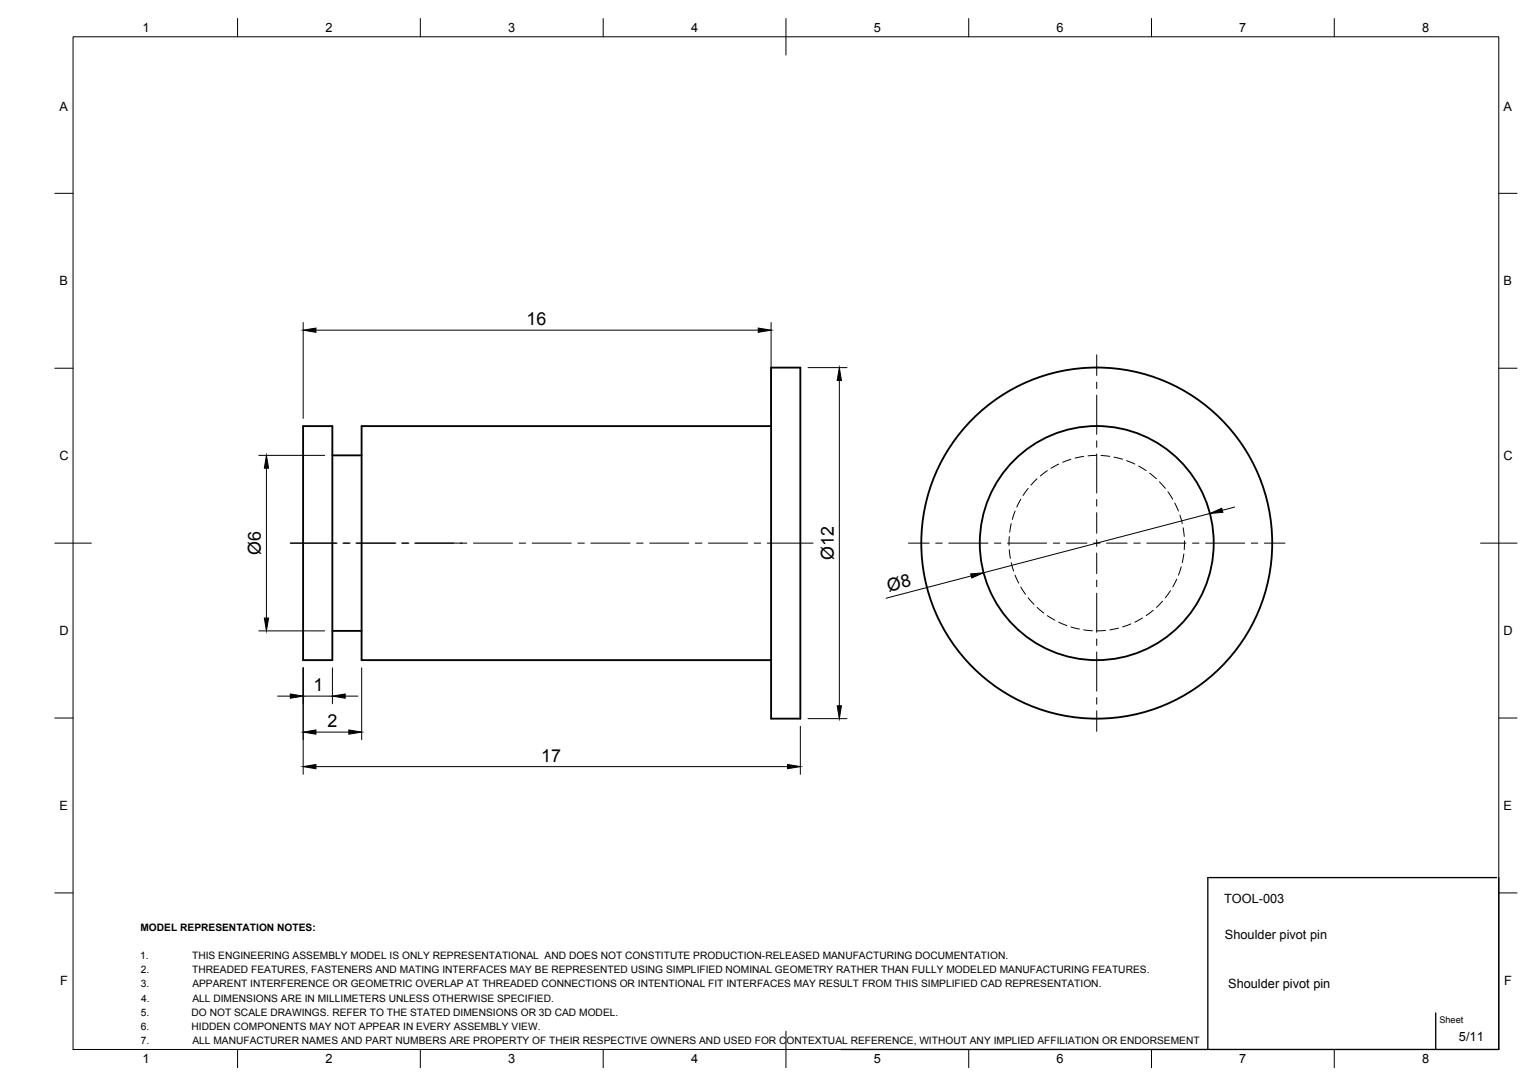
ISO-10303-21;
HEADER;
/* Generated by software containing ST-Developer
 * from STEP Tools, Inc. (www.steptools.com) 
 */

FILE_DESCRIPTION(
/* description */ (''),
/* implementation_level */ '2;1');

FILE_NAME(
/* name */ 'Shoulder pivot pin.step',
/* time_stamp */ '2026-11-10T05:20:16-08:00',
/* author */ (''),
/* organization */ (''),
/* preprocessor_version */ 'ST-DEVELOPER v20.2',
/* originating_system */ 'Autodesk Translation Framework v15.17.0.0',
/* authorisation */ '');

FILE_SCHEMA (('AUTOMOTIVE_DESIGN { 1 0 10303 214 3 1 1 }'));
ENDSEC;

DATA;
#10=MECHANICAL_DESIGN_GEOMETRIC_PRESENTATION_REPRESENTATION('',(#114),#24809);
#94=SHAPE_REPRESENTATION_RELATIONSHIP('SRR','None',#24857,#104);
#104=ADVANCED_BREP_SHAPE_REPRESENTATION('',(#124),#24800);
#114=STYLED_ITEM('',(#24920),#124);
#124=MANIFOLD_SOLID_BREP('Body1',#9891);
#144=FACE_BOUND('',#2081,.T.);
#145=FACE_BOUND('',#2083,.T.);
#146=FACE_BOUND('',#2086,.T.);
#1187=PLANE('',#10235);
#1188=PLANE('',#10237);
#1189=PLANE('',#10241);
#1190=PLANE('',#10246);
#1191=PLANE('',#10248);
#1514=FACE_OUTER_BOUND('',#2079,.T.);
#1515=FACE_OUTER_BOUND('',#2080,.T.);
#1516=FACE_OUTER_BOUND('',#2082,.T.);
#1517=FACE_OUTER_BOUND('',#2084,.T.);
#1518=FACE_OUTER_BOUND('',#2085,.T.);
#1519=FACE_OUTER_BOUND('',#2087,.T.);
#1520=FACE_OUTER_BOUND('',#2088,.T.);
#1521=FACE_OUTER_BOUND('',#2089,.T.);
#1522=FACE_OUTER_BOUND('',#2090,.T.);
#2079=EDGE_LOOP('',(#7449,#7450,#7451,#7452));
#2080=EDGE_LOOP('',(#7453));
#2081=EDGE_LOOP('',(#7454));
#2082=EDGE_LOOP('',(#7455));
#2083=EDGE_LOOP('',(#7456));
#2084=EDGE_LOOP('',(#7457,#7458,#7459,#7460));
#2085=EDGE_LOOP('',(#7461));
#2086=EDGE_LOOP('',(#7462));
#2087=EDGE_LOOP('',(#7463,#7464,#7465,#7466));
#2088=EDGE_LOOP('',(#7467));
#2089=EDGE_LOOP('',(#7468,#7469,#7470,#7471));
#2090=EDGE_LOOP('',(#7472));
#2727=LINE('',#14885,#3315);
#2728=LINE('',#14896,#3316);
#2729=LINE('',#14904,#3317);
#2730=LINE('',#14908,#3318);
#3315=VECTOR('',#11365,0.3);
#3316=VECTOR('',#11380,0.4);
#3317=VECTOR('',#11389,0.6);
#3318=VECTOR('',#11396,0.4);
#3679=CIRCLE('',#10233,0.3);
#3680=CIRCLE('',#10234,0.3);
#3681=CIRCLE('',#10236,0.4);
#3682=CIRCLE('',#10238,0.4);
#3683=CIRCLE('',#10240,0.4);
#3684=CIRCLE('',#10242,0.6);
#3685=CIRCLE('',#10243,0.4);
#3686=CIRCLE('',#10245,0.6);
#4223=VERTEX_POINT('',#14882);
#4224=VERTEX_POINT('',#14884);
#4225=VERTEX_POINT('',#14888);
#4226=VERTEX_POINT('',#14891);
#4227=VERTEX_POINT('',#14894);
#4228=VERTEX_POINT('',#14898);
#4229=VERTEX_POINT('',#14900);
#4230=VERTEX_POINT('',#14903);
#5383=EDGE_CURVE('',#4223,#4223,#3679,.T.);
#5384=EDGE_CURVE('',#4223,#4224,#2727,.T.);
#5385=EDGE_CURVE('',#4224,#4224,#3680,.T.);
#5386=EDGE_CURVE('',#4225,#4225,#3681,.T.);
#5387=EDGE_CURVE('',#4226,#4226,#3682,.T.);
#5388=EDGE_CURVE('',#4227,#4227,#3683,.T.);
#5389=EDGE_CURVE('',#4227,#4226,#2728,.T.);
#5390=EDGE_CURVE('',#4228,#4228,#3684,.T.);
#5391=EDGE_CURVE('',#4229,#4229,#3685,.T.);
#5392=EDGE_CURVE('',#4228,#4230,#2729,.T.);
#5393=EDGE_CURVE('',#4230,#4230,#3686,.T.);
#5394=EDGE_CURVE('',#4225,#4229,#2730,.T.);
#7449=ORIENTED_EDGE('',*,*,#5383,.T.);
#7450=ORIENTED_EDGE('',*,*,#5384,.T.);
#7451=ORIENTED_EDGE('',*,*,#5385,.F.);
#7452=ORIENTED_EDGE('',*,*,#5384,.F.);
#7453=ORIENTED_EDGE('',*,*,#5386,.F.);
#7454=ORIENTED_EDGE('',*,*,#5383,.F.);
#7455=ORIENTED_EDGE('',*,*,#5387,.F.);
#7456=ORIENTED_EDGE('',*,*,#5385,.T.);
#7457=ORIENTED_EDGE('',*,*,#5388,.F.);
#7458=ORIENTED_EDGE('',*,*,#5389,.T.);
#7459=ORIENTED_EDGE('',*,*,#5387,.T.);
#7460=ORIENTED_EDGE('',*,*,#5389,.F.);
#7461=ORIENTED_EDGE('',*,*,#5390,.T.);
#7462=ORIENTED_EDGE('',*,*,#5391,.F.);
#7463=ORIENTED_EDGE('',*,*,#5390,.F.);
#7464=ORIENTED_EDGE('',*,*,#5392,.T.);
#7465=ORIENTED_EDGE('',*,*,#5393,.T.);
#7466=ORIENTED_EDGE('',*,*,#5392,.F.);
#7467=ORIENTED_EDGE('',*,*,#5393,.F.);
#7468=ORIENTED_EDGE('',*,*,#5386,.T.);
#7469=ORIENTED_EDGE('',*,*,#5394,.T.);
#7470=ORIENTED_EDGE('',*,*,#5391,.T.);
#7471=ORIENTED_EDGE('',*,*,#5394,.F.);
#7472=ORIENTED_EDGE('',*,*,#5388,.T.);
#9207=CYLINDRICAL_SURFACE('',#10232,0.3);
#9208=CYLINDRICAL_SURFACE('',#10239,0.4);
#9209=CYLINDRICAL_SURFACE('',#10244,0.6);
#9210=CYLINDRICAL_SURFACE('',#10247,0.4);
#9540=ADVANCED_FACE('',(#1514),#9207,.T.);
#9541=ADVANCED_FACE('',(#1515,#144),#1187,.F.);
#9542=ADVANCED_FACE('',(#1516,#145),#1188,.F.);
#9543=ADVANCED_FACE('',(#1517),#9208,.T.);
#9544=ADVANCED_FACE('',(#1518,#146),#1189,.T.);
#9545=ADVANCED_FACE('',(#1519),#9209,.T.);
#9546=ADVANCED_FACE('',(#1520),#1190,.F.);
#9547=ADVANCED_FACE('',(#1521),#9210,.T.);
#9548=ADVANCED_FACE('',(#1522),#1191,.T.);
#9891=CLOSED_SHELL('',(#9540,#9541,#9542,#9543,#9544,#9545,#9546,#9547,
#9548));
#10231=AXIS2_PLACEMENT_3D('',#14880,#11359,#11360);
#10232=AXIS2_PLACEMENT_3D('',#14881,#11361,#11362);
#10233=AXIS2_PLACEMENT_3D('',#14883,#11363,#11364);
#10234=AXIS2_PLACEMENT_3D('',#14886,#11366,#11367);
#10235=AXIS2_PLACEMENT_3D('',#14887,#11368,#11369);
#10236=AXIS2_PLACEMENT_3D('',#14889,#11370,#11371);
#10237=AXIS2_PLACEMENT_3D('',#14890,#11372,#11373);
#10238=AXIS2_PLACEMENT_3D('',#14892,#11374,#11375);
#10239=AXIS2_PLACEMENT_3D('',#14893,#11376,#11377);
#10240=AXIS2_PLACEMENT_3D('',#14895,#11378,#11379);
#10241=AXIS2_PLACEMENT_3D('',#14897,#11381,#11382);
#10242=AXIS2_PLACEMENT_3D('',#14899,#11383,#11384);
#10243=AXIS2_PLACEMENT_3D('',#14901,#11385,#11386);
#10244=AXIS2_PLACEMENT_3D('',#14902,#11387,#11388);
#10245=AXIS2_PLACEMENT_3D('',#14905,#11390,#11391);
#10246=AXIS2_PLACEMENT_3D('',#14906,#11392,#11393);
#10247=AXIS2_PLACEMENT_3D('',#14907,#11394,#11395);
#10248=AXIS2_PLACEMENT_3D('',#14909,#11397,#11398);
#11359=DIRECTION('axis',(0.,0.,1.));
#11360=DIRECTION('refdir',(1.,0.,0.));
#11361=DIRECTION('center_axis',(0.,0.,1.));
#11362=DIRECTION('ref_axis',(1.,0.,0.));
#11363=DIRECTION('center_axis',(0.,0.,1.));
#11364=DIRECTION('ref_axis',(1.,0.,0.));
#11365=DIRECTION('',(0.,0.,1.));
#11366=DIRECTION('center_axis',(0.,0.,1.));
#11367=DIRECTION('ref_axis',(1.,0.,0.));
#11368=DIRECTION('center_axis',(0.,0.,-1.));
#11369=DIRECTION('ref_axis',(-1.,0.,0.));
#11370=DIRECTION('center_axis',(0.,0.,-1.));
#11371=DIRECTION('ref_axis',(1.,0.,0.));
#11372=DIRECTION('center_axis',(0.,0.,1.));
#11373=DIRECTION('ref_axis',(1.,0.,0.));
#11374=DIRECTION('center_axis',(0.,0.,1.));
#11375=DIRECTION('ref_axis',(1.,0.,0.));
#11376=DIRECTION('center_axis',(0.,0.,1.));
#11377=DIRECTION('ref_axis',(1.,0.,0.));
#11378=DIRECTION('center_axis',(0.,0.,1.));
#11379=DIRECTION('ref_axis',(1.,0.,0.));
#11380=DIRECTION('',(0.,0.,-1.));
#11381=DIRECTION('center_axis',(0.,0.,1.));
#11382=DIRECTION('ref_axis',(1.,0.,0.));
#11383=DIRECTION('center_axis',(0.,0.,1.));
#11384=DIRECTION('ref_axis',(1.,0.,0.));
#11385=DIRECTION('center_axis',(0.,0.,1.));
#11386=DIRECTION('ref_axis',(1.,0.,0.));
#11387=DIRECTION('center_axis',(0.,0.,1.));
#11388=DIRECTION('ref_axis',(1.,0.,0.));
#11389=DIRECTION('',(0.,0.,-1.));
#11390=DIRECTION('center_axis',(0.,0.,1.));
#11391=DIRECTION('ref_axis',(1.,0.,0.));
#11392=DIRECTION('center_axis',(0.,0.,1.));
#11393=DIRECTION('ref_axis',(1.,0.,0.));
#11394=DIRECTION('center_axis',(0.,0.,1.));
#11395=DIRECTION('ref_axis',(1.,0.,0.));
#11396=DIRECTION('',(0.,0.,-1.));
#11397=DIRECTION('center_axis',(0.,0.,1.));
#11398=DIRECTION('ref_axis',(1.,0.,0.));
#14880=CARTESIAN_POINT('',(0.,0.,0.));
#14881=CARTESIAN_POINT('Origin',(0.,0.,0.75));
#14882=CARTESIAN_POINT('',(-0.3,-3.67394039744206E-17,0.7));
#14883=CARTESIAN_POINT('Origin',(0.,0.,0.7));
#14884=CARTESIAN_POINT('',(-0.3,-3.67394039744206E-17,0.8));
#14885=CARTESIAN_POINT('',(-0.3,-3.67394039744206E-17,0.75));
#14886=CARTESIAN_POINT('Origin',(0.,0.,0.8));
#14887=CARTESIAN_POINT('Origin',(0.7,0.,0.7));
#14888=CARTESIAN_POINT('',(-0.4,4.89858719658941E-17,0.7));
#14889=CARTESIAN_POINT('Origin',(0.,0.,0.7));
#14890=CARTESIAN_POINT('Origin',(0.3,0.,0.8));
#14891=CARTESIAN_POINT('',(-0.4,-4.89858719658941E-17,0.8));
#14892=CARTESIAN_POINT('Origin',(0.,0.,0.8));
#14893=CARTESIAN_POINT('Origin',(0.,0.,-0.7));
#14894=CARTESIAN_POINT('',(-0.4,-4.89858719658941E-17,0.9));
#14895=CARTESIAN_POINT('Origin',(0.,0.,0.9));
#14896=CARTESIAN_POINT('',(-0.4,-4.89858719658941E-17,-0.7));
#14897=CARTESIAN_POINT('Origin',(0.,0.,-0.7));
#14898=CARTESIAN_POINT('',(-0.6,-7.34788079488412E-17,-0.7));
#14899=CARTESIAN_POINT('Origin',(0.,0.,-0.7));
#14900=CARTESIAN_POINT('',(-0.4,-4.89858719658941E-17,-0.7));
#14901=CARTESIAN_POINT('Origin',(0.,0.,-0.7));
#14902=CARTESIAN_POINT('Origin',(0.,0.,-0.8));
#14903=CARTESIAN_POINT('',(-0.6,-7.34788079488412E-17,-0.8));
#14904=CARTESIAN_POINT('',(-0.6,-7.34788079488412E-17,-0.8));
#14905=CARTESIAN_POINT('Origin',(0.,0.,-0.8));
#14906=CARTESIAN_POINT('Origin',(0.,0.,-0.8));
#14907=CARTESIAN_POINT('Origin',(0.,0.,-0.7));
#14908=CARTESIAN_POINT('',(-0.4,-4.89858719658941E-17,-0.7));
#14909=CARTESIAN_POINT('Origin',(0.,0.,0.9));
#24787=UNCERTAINTY_MEASURE_WITH_UNIT(LENGTH_MEASURE(0.001),#24810,
'DISTANCE_ACCURACY_VALUE',
'Maximum model space distance between geometric entities at asserted c
onnectivities');
#24796=UNCERTAINTY_MEASURE_WITH_UNIT(LENGTH_MEASURE(0.001),#24810,
'DISTANCE_ACCURACY_VALUE',
'Maximum model space distance between geometric entities at asserted c
onnectivities');
#24800=(
GEOMETRIC_REPRESENTATION_CONTEXT(3)
GLOBAL_UNCERTAINTY_ASSIGNED_CONTEXT((#24787))
GLOBAL_UNIT_ASSIGNED_CONTEXT((#24810,#24812,#24813))
REPRESENTATION_CONTEXT('','3D')
);
#24809=(
GEOMETRIC_REPRESENTATION_CONTEXT(3)
GLOBAL_UNCERTAINTY_ASSIGNED_CONTEXT((#24796))
GLOBAL_UNIT_ASSIGNED_CONTEXT((#24810,#24812,#24813))
REPRESENTATION_CONTEXT('','3D')
);
#24810=(
LENGTH_UNIT()
NAMED_UNIT(*)
SI_UNIT(.CENTI.,.METRE.)
);
#24812=(
NAMED_UNIT(*)
PLANE_ANGLE_UNIT()
SI_UNIT($,.RADIAN.)
);
#24813=(
NAMED_UNIT(*)
SI_UNIT($,.STERADIAN.)
SOLID_ANGLE_UNIT()
);
#24817=SHAPE_DEFINITION_REPRESENTATION(#24829,#24857);
#24829=PRODUCT_DEFINITION_SHAPE('',$,#24870);
#24857=SHAPE_REPRESENTATION('',(#10231),#24800);
#24866=PRODUCT_DEFINITION_CONTEXT('part definition',#24904,'design');
#24870=PRODUCT_DEFINITION('Shoulder pivot pin','Shoulder pivot pin',#24882,
#24866);
#24882=PRODUCT_DEFINITION_FORMATION('',$,#24909);
#24904=APPLICATION_CONTEXT(
'Core Data for Automotive Mechanical Design Process');
#24905=PRODUCT_CONTEXT('part definition',#24904,'mechanical');
#24909=PRODUCT('Shoulder pivot pin','Shoulder pivot pin',$,(#24905));
#24920=PRESENTATION_STYLE_ASSIGNMENT((#24928));
#24928=SURFACE_STYLE_USAGE(.BOTH.,#24936);
#24936=SURFACE_SIDE_STYLE('',(#24944));
#24944=SURFACE_STYLE_FILL_AREA(#24952);
#24952=FILL_AREA_STYLE('Pivot dark gray',(#24960));
#24960=FILL_AREA_STYLE_COLOUR('Pivot dark gray',#24968);
#24968=COLOUR_RGB('Pivot dark gray',0.27843137254902,0.309803921568627,
0.352941176470588);
ENDSEC;
END-ISO-10303-21;
